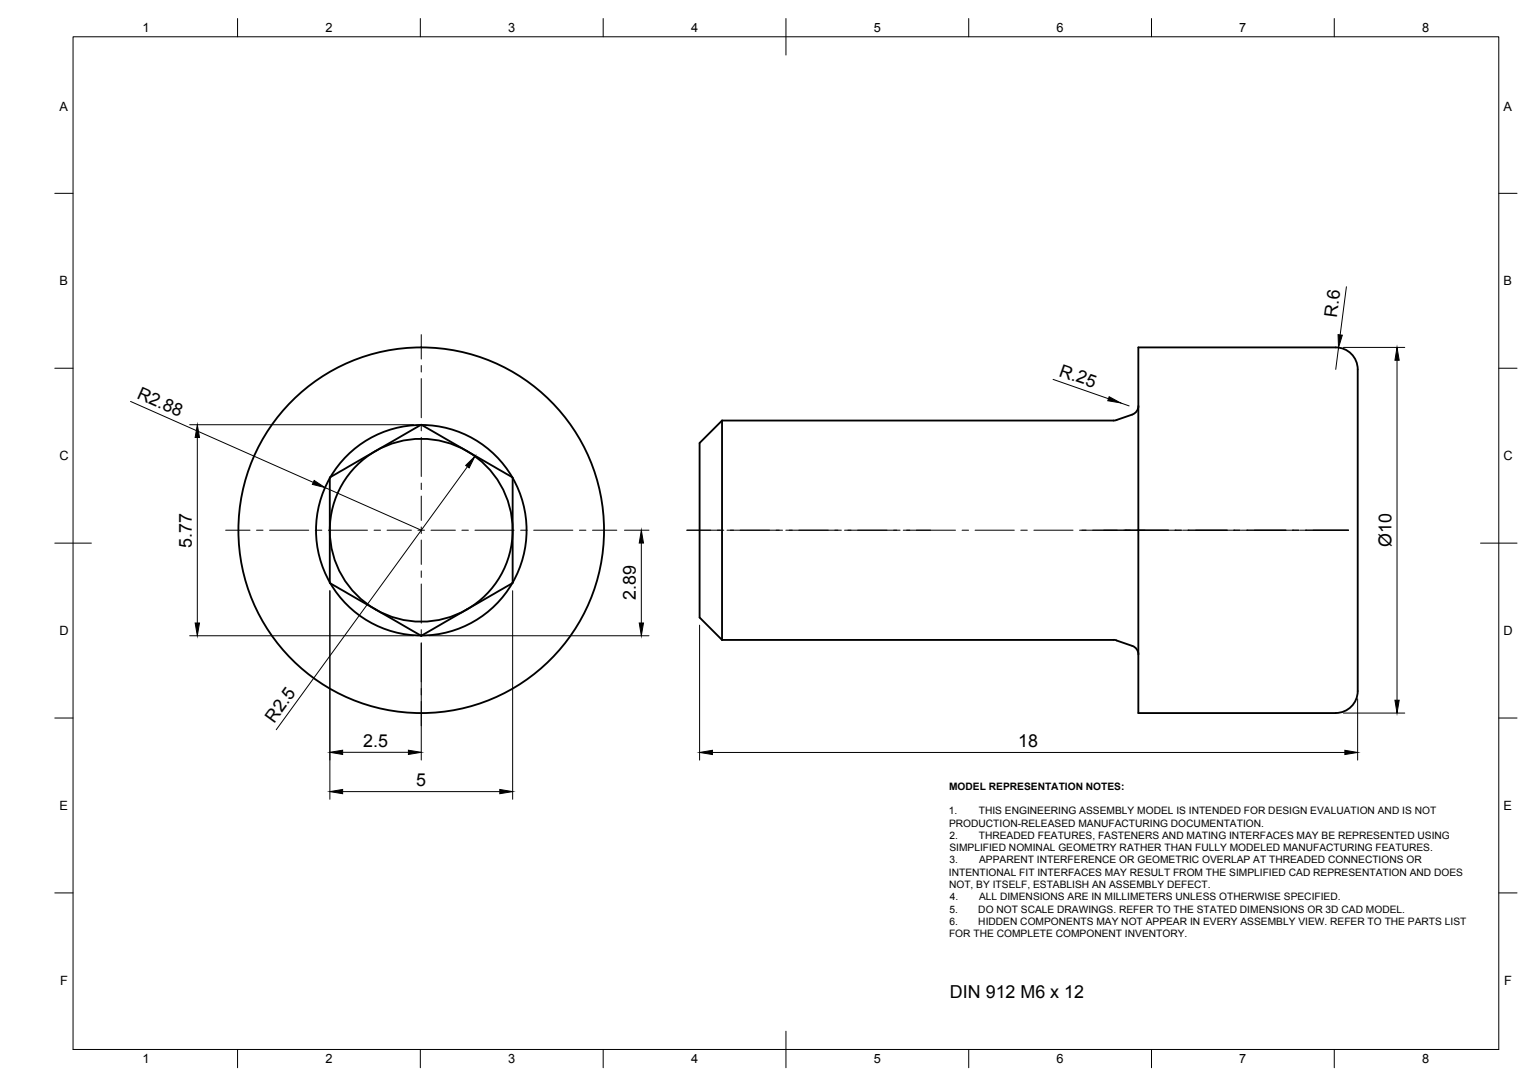
ISO-10303-21;
HEADER;
/* Generated by software containing ST-Developer
 * from STEP Tools, Inc. (www.steptools.com) 
 */

FILE_DESCRIPTION(
/* description */ ('STEP AP214'),
/* implementation_level */ '2;1');

FILE_NAME(
/* name */ 'DIN 912 M6x12.step',
/* time_stamp */ '2026-10-07T12:18:07-07:00',
/* author */ (''),
/* organization */ (''),
/* preprocessor_version */ 'ST-DEVELOPER v20.2',
/* originating_system */ 'Autodesk Translation Framework v15.15.0.0',
/* authorisation */ '');

FILE_SCHEMA (('AUTOMOTIVE_DESIGN { 1 0 10303 214 3 1 1 }'));
ENDSEC;

DATA;
#10=MECHANICAL_DESIGN_GEOMETRIC_PRESENTATION_REPRESENTATION('',(#133),#62974);
#73=(
BOUNDED_CURVE()
B_SPLINE_CURVE(2,(#62798,#62799,#62800),.UNSPECIFIED.,.F.,.F.)
B_SPLINE_CURVE_WITH_KNOTS((3,3),(-0.604448710450841,-0.208150383555822),
 .UNSPECIFIED.)
CURVE()
GEOMETRIC_REPRESENTATION_ITEM()
RATIONAL_B_SPLINE_CURVE((1.32194252928783,1.52287779373958,1.32194252928783))
REPRESENTATION_ITEM('')
);
#74=(
BOUNDED_CURVE()
B_SPLINE_CURVE(2,(#62844,#62845,#62846),.UNSPECIFIED.,.F.,.F.)
B_SPLINE_CURVE_WITH_KNOTS((3,3),(0.208150383555825,0.60444871045084),
 .UNSPECIFIED.)
CURVE()
GEOMETRIC_REPRESENTATION_ITEM()
RATIONAL_B_SPLINE_CURVE((1.32194252928783,1.52287779373957,1.32194252928783))
REPRESENTATION_ITEM('')
);
#75=(
BOUNDED_CURVE()
B_SPLINE_CURVE(2,(#62851,#62852,#62853),.UNSPECIFIED.,.F.,.F.)
B_SPLINE_CURVE_WITH_KNOTS((3,3),(0.208150383555826,0.604448710450838),
 .UNSPECIFIED.)
CURVE()
GEOMETRIC_REPRESENTATION_ITEM()
RATIONAL_B_SPLINE_CURVE((1.32194252928783,1.52287779373957,1.32194252928783))
REPRESENTATION_ITEM('')
);
#76=(
BOUNDED_CURVE()
B_SPLINE_CURVE(2,(#62858,#62859,#62860),.UNSPECIFIED.,.F.,.F.)
B_SPLINE_CURVE_WITH_KNOTS((3,3),(0.208150383555825,0.60444871045084),
 .UNSPECIFIED.)
CURVE()
GEOMETRIC_REPRESENTATION_ITEM()
RATIONAL_B_SPLINE_CURVE((1.32194252928783,1.52287779373957,1.32194252928783))
REPRESENTATION_ITEM('')
);
#77=(
BOUNDED_CURVE()
B_SPLINE_CURVE(2,(#62869,#62870,#62871),.UNSPECIFIED.,.F.,.F.)
B_SPLINE_CURVE_WITH_KNOTS((3,3),(0.208150383555823,0.604448710450839),
 .UNSPECIFIED.)
CURVE()
GEOMETRIC_REPRESENTATION_ITEM()
RATIONAL_B_SPLINE_CURVE((1.32194252928783,1.52287779373958,1.32194252928783))
REPRESENTATION_ITEM('')
);
#78=(
BOUNDED_CURVE()
B_SPLINE_CURVE(2,(#62876,#62877,#62878),.UNSPECIFIED.,.F.,.F.)
B_SPLINE_CURVE_WITH_KNOTS((3,3),(0.208150383555823,0.604448710450836),
 .UNSPECIFIED.)
CURVE()
GEOMETRIC_REPRESENTATION_ITEM()
RATIONAL_B_SPLINE_CURVE((1.32194252928783,1.52287779373958,1.32194252928783))
REPRESENTATION_ITEM('')
);
#109=SHAPE_REPRESENTATION_RELATIONSHIP('SRR','None',#63032,#121);
#121=ADVANCED_BREP_SHAPE_REPRESENTATION('',(#145),#62973);
#133=STYLED_ITEM('',(#63090),#145);
#145=MANIFOLD_SOLID_BREP('Body1',#15203);
#277=FACE_BOUND('',#5497,.T.);
#278=FACE_BOUND('',#5507,.T.);
#720=PLANE('',#16916);
#721=PLANE('',#16923);
#722=PLANE('',#16928);
#723=PLANE('',#16929);
#724=PLANE('',#16930);
#725=PLANE('',#16931);
#726=PLANE('',#16932);
#727=PLANE('',#16933);
#728=PLANE('',#16934);
#729=PLANE('',#16935);
#730=PLANE('',#16936);
#731=PLANE('',#16937);
#732=PLANE('',#16938);
#733=PLANE('',#16939);
#734=PLANE('',#16940);
#1048=CONICAL_SURFACE('',#16885,2.5,1.04719755119659);
#1049=CONICAL_SURFACE('',#16892,2.88,1.04719755119651);
#1050=CONICAL_SURFACE('',#16913,3.,0.785398163397449);
#1051=CONICAL_SURFACE('',#16915,3.0139499546386,0.335638550327472);
#1052=CONICAL_SURFACE('',#16917,2.88,1.04719755119651);
#1053=CONICAL_SURFACE('',#16919,2.88,1.04719755119651);
#1054=CONICAL_SURFACE('',#16921,2.88,1.04719755119651);
#1055=CONICAL_SURFACE('',#16924,2.88,1.04719755119651);
#1056=CONICAL_SURFACE('',#16926,2.88,1.04719755119651);
#2215=LINE('',#62783,#3408);
#2216=LINE('',#62812,#3409);
#2217=LINE('',#62824,#3410);
#2218=LINE('',#62836,#3411);
#2219=LINE('',#62839,#3412);
#2220=LINE('',#62864,#3413);
#2221=LINE('',#62865,#3414);
#2222=LINE('',#62882,#3415);
#2223=LINE('',#62883,#3416);
#2224=LINE('',#62886,#3417);
#2225=LINE('',#62887,#3418);
#2226=LINE('',#62891,#3419);
#2227=LINE('',#62892,#3420);
#2228=LINE('',#62894,#3421);
#2229=LINE('',#62895,#3422);
#2230=LINE('',#62897,#3423);
#2231=LINE('',#62899,#3424);
#2232=LINE('',#62900,#3425);
#2233=LINE('',#62902,#3426);
#2234=LINE('',#62904,#3427);
#2235=LINE('',#62906,#3428);
#2236=LINE('',#62907,#3429);
#2237=LINE('',#62909,#3430);
#2238=LINE('',#62910,#3431);
#2239=LINE('',#62912,#3432);
#2240=LINE('',#62914,#3433);
#2241=LINE('',#62915,#3434);
#2242=LINE('',#62918,#3435);
#2243=LINE('',#62920,#3436);
#2244=LINE('',#62921,#3437);
#2245=LINE('',#62922,#3438);
#2246=LINE('',#62924,#3439);
#2247=LINE('',#62925,#3440);
#2248=LINE('',#62926,#3441);
#2249=LINE('',#62927,#3442);
#3408=VECTOR('',#21212,2.5);
#3409=VECTOR('',#21241,5.);
#3410=VECTOR('',#21256,3.);
#3411=VECTOR('',#21271,3.);
#3412=VECTOR('',#21276,3.0139499546386);
#3413=VECTOR('',#21293,1000.);
#3414=VECTOR('',#21294,1000.);
#3415=VECTOR('',#21305,1000.);
#3416=VECTOR('',#21306,1000.);
#3417=VECTOR('',#21309,1000.);
#3418=VECTOR('',#21310,1000.);
#3419=VECTOR('',#21315,1000.);
#3420=VECTOR('',#21316,1000.);
#3421=VECTOR('',#21317,1000.);
#3422=VECTOR('',#21318,1000.);
#3423=VECTOR('',#21321,1000.);
#3424=VECTOR('',#21322,1000.);
#3425=VECTOR('',#21323,1000.);
#3426=VECTOR('',#21326,1000.);
#3427=VECTOR('',#21327,1000.);
#3428=VECTOR('',#21328,1000.);
#3429=VECTOR('',#21329,1000.);
#3430=VECTOR('',#21332,1000.);
#3431=VECTOR('',#21333,1000.);
#3432=VECTOR('',#21334,1000.);
#3433=VECTOR('',#21335,1000.);
#3434=VECTOR('',#21336,1000.);
#3435=VECTOR('',#21339,1000.);
#3436=VECTOR('',#21340,1000.);
#3437=VECTOR('',#21341,1000.);
#3438=VECTOR('',#21342,1000.);
#3439=VECTOR('',#21345,1000.);
#3440=VECTOR('',#21346,1000.);
#3441=VECTOR('',#21347,1000.);
#3442=VECTOR('',#21348,1000.);
#3688=CYLINDRICAL_SURFACE('',#16899,5.);
#3689=CYLINDRICAL_SURFACE('',#16906,3.);
#4528=FACE_OUTER_BOUND('',#5478,.T.);
#4529=FACE_OUTER_BOUND('',#5479,.T.);
#4530=FACE_OUTER_BOUND('',#5480,.T.);
#4531=FACE_OUTER_BOUND('',#5481,.T.);
#4532=FACE_OUTER_BOUND('',#5482,.T.);
#4533=FACE_OUTER_BOUND('',#5483,.T.);
#4534=FACE_OUTER_BOUND('',#5484,.T.);
#4535=FACE_OUTER_BOUND('',#5485,.T.);
#4536=FACE_OUTER_BOUND('',#5486,.T.);
#4537=FACE_OUTER_BOUND('',#5487,.T.);
#4538=FACE_OUTER_BOUND('',#5488,.T.);
#4539=FACE_OUTER_BOUND('',#5489,.T.);
#4540=FACE_OUTER_BOUND('',#5490,.T.);
#4541=FACE_OUTER_BOUND('',#5491,.T.);
#4542=FACE_OUTER_BOUND('',#5492,.T.);
#4543=FACE_OUTER_BOUND('',#5493,.T.);
#4544=FACE_OUTER_BOUND('',#5494,.T.);
#4545=FACE_OUTER_BOUND('',#5495,.T.);
#4546=FACE_OUTER_BOUND('',#5496,.T.);
#4547=FACE_OUTER_BOUND('',#5498,.T.);
#4548=FACE_OUTER_BOUND('',#5499,.T.);
#4549=FACE_OUTER_BOUND('',#5500,.T.);
#4550=FACE_OUTER_BOUND('',#5501,.T.);
#4551=FACE_OUTER_BOUND('',#5502,.T.);
#4552=FACE_OUTER_BOUND('',#5503,.T.);
#4553=FACE_OUTER_BOUND('',#5504,.T.);
#4554=FACE_OUTER_BOUND('',#5505,.T.);
#4555=FACE_OUTER_BOUND('',#5506,.T.);
#4556=FACE_OUTER_BOUND('',#5508,.T.);
#5478=EDGE_LOOP('',(#14117,#14118,#14119,#14120,#14121,#14122,#14123,#14124));
#5479=EDGE_LOOP('',(#14125,#14126));
#5480=EDGE_LOOP('',(#14127,#14128,#14129,#14130,#14131));
#5481=EDGE_LOOP('',(#14132,#14133,#14134,#14135,#14136));
#5482=EDGE_LOOP('',(#14137,#14138,#14139,#14140,#14141));
#5483=EDGE_LOOP('',(#14142,#14143,#14144,#14145,#14146,#14147));
#5484=EDGE_LOOP('',(#14148,#14149,#14150,#14151));
#5485=EDGE_LOOP('',(#14152,#14153,#14154,#14155,#14156));
#5486=EDGE_LOOP('',(#14157,#14158,#14159,#14160));
#5487=EDGE_LOOP('',(#14161));
#5488=EDGE_LOOP('',(#14162,#14163));
#5489=EDGE_LOOP('',(#14164,#14165));
#5490=EDGE_LOOP('',(#14166,#14167));
#5491=EDGE_LOOP('',(#14168,#14169,#14170));
#5492=EDGE_LOOP('',(#14171,#14172));
#5493=EDGE_LOOP('',(#14173,#14174));
#5494=EDGE_LOOP('',(#14175,#14176,#14177));
#5495=EDGE_LOOP('',(#14178,#14179,#14180));
#5496=EDGE_LOOP('',(#14181));
#5497=EDGE_LOOP('',(#14182));
#5498=EDGE_LOOP('',(#14183,#14184,#14185,#14186,#14187,#14188,#14189));
#5499=EDGE_LOOP('',(#14190,#14191,#14192,#14193,#14194,#14195,#14196));
#5500=EDGE_LOOP('',(#14197,#14198,#14199,#14200,#14201,#14202,#14203));
#5501=EDGE_LOOP('',(#14204,#14205,#14206,#14207,#14208,#14209,#14210));
#5502=EDGE_LOOP('',(#14211,#14212,#14213,#14214,#14215,#14216,#14217));
#5503=EDGE_LOOP('',(#14218,#14219,#14220,#14221,#14222,#14223,#14224));
#5504=EDGE_LOOP('',(#14225,#14226,#14227));
#5505=EDGE_LOOP('',(#14228,#14229,#14230));
#5506=EDGE_LOOP('',(#14231));
#5507=EDGE_LOOP('',(#14232,#14233,#14234,#14235,#14236,#14237,#14238,#14239,
#14240,#14241,#14242,#14243,#14244,#14245,#14246,#14247,#14248,#14249));
#5508=EDGE_LOOP('',(#14250,#14251,#14252));
#6194=CIRCLE('',#16886,2.5);
#6195=CIRCLE('',#16887,2.5);
#6196=CIRCLE('',#16888,2.5);
#6197=CIRCLE('',#16889,2.5);
#6198=CIRCLE('',#16890,2.5);
#6199=CIRCLE('',#16891,2.5);
#6200=CIRCLE('',#16893,2.88);
#6201=CIRCLE('',#16895,4.4);
#6202=CIRCLE('',#16896,0.600000000000098);
#6203=CIRCLE('',#16897,5.);
#6204=CIRCLE('',#16898,5.);
#6205=CIRCLE('',#16900,5.);
#6206=CIRCLE('',#16902,3.0139499546386);
#6207=CIRCLE('',#16903,0.249999999998187);
#6208=CIRCLE('',#16904,3.);
#6209=CIRCLE('',#16905,3.);
#6210=CIRCLE('',#16907,3.);
#6211=CIRCLE('',#16908,3.);
#6212=CIRCLE('',#16910,3.4);
#6213=CIRCLE('',#16911,0.249999999999786);
#6214=CIRCLE('',#16912,3.1639499546386);
#6215=CIRCLE('',#16914,2.3865);
#6216=CIRCLE('',#16918,2.88);
#6217=CIRCLE('',#16920,2.88);
#6218=CIRCLE('',#16922,2.88);
#6219=CIRCLE('',#16925,2.88);
#6220=CIRCLE('',#16927,2.88);
#7580=VERTEX_POINT('',#62781);
#7581=VERTEX_POINT('',#62782);
#7582=VERTEX_POINT('',#62784);
#7583=VERTEX_POINT('',#62786);
#7584=VERTEX_POINT('',#62788);
#7585=VERTEX_POINT('',#62790);
#7586=VERTEX_POINT('',#62792);
#7587=VERTEX_POINT('',#62796);
#7588=VERTEX_POINT('',#62797);
#7589=VERTEX_POINT('',#62803);
#7590=VERTEX_POINT('',#62805);
#7591=VERTEX_POINT('',#62807);
#7592=VERTEX_POINT('',#62811);
#7593=VERTEX_POINT('',#62815);
#7594=VERTEX_POINT('',#62817);
#7595=VERTEX_POINT('',#62819);
#7596=VERTEX_POINT('',#62823);
#7597=VERTEX_POINT('',#62825);
#7598=VERTEX_POINT('',#62829);
#7599=VERTEX_POINT('',#62831);
#7600=VERTEX_POINT('',#62835);
#7601=VERTEX_POINT('',#62842);
#7602=VERTEX_POINT('',#62843);
#7603=VERTEX_POINT('',#62849);
#7604=VERTEX_POINT('',#62850);
#7605=VERTEX_POINT('',#62856);
#7606=VERTEX_POINT('',#62857);
#7607=VERTEX_POINT('',#62863);
#7608=VERTEX_POINT('',#62867);
#7609=VERTEX_POINT('',#62868);
#7610=VERTEX_POINT('',#62874);
#7611=VERTEX_POINT('',#62875);
#7612=VERTEX_POINT('',#62881);
#7613=VERTEX_POINT('',#62885);
#7614=VERTEX_POINT('',#62890);
#7615=VERTEX_POINT('',#62893);
#7616=VERTEX_POINT('',#62898);
#7617=VERTEX_POINT('',#62903);
#7618=VERTEX_POINT('',#62905);
#7619=VERTEX_POINT('',#62911);
#7620=VERTEX_POINT('',#62913);
#7621=VERTEX_POINT('',#62917);
#7622=VERTEX_POINT('',#62919);
#9765=EDGE_CURVE('',#7580,#7581,#2215,.T.);
#9766=EDGE_CURVE('',#7582,#7581,#6194,.T.);
#9767=EDGE_CURVE('',#7583,#7582,#6195,.T.);
#9768=EDGE_CURVE('',#7584,#7583,#6196,.T.);
#9769=EDGE_CURVE('',#7585,#7584,#6197,.T.);
#9770=EDGE_CURVE('',#7586,#7585,#6198,.T.);
#9771=EDGE_CURVE('',#7581,#7586,#6199,.T.);
#9772=EDGE_CURVE('',#7587,#7588,#73,.F.);
#9773=EDGE_CURVE('',#7587,#7588,#6200,.T.);
#9774=EDGE_CURVE('',#7589,#7589,#6201,.T.);
#9775=EDGE_CURVE('',#7589,#7590,#6202,.T.);
#9776=EDGE_CURVE('',#7590,#7591,#6203,.T.);
#9777=EDGE_CURVE('',#7591,#7590,#6204,.T.);
#9778=EDGE_CURVE('',#7591,#7592,#2216,.T.);
#9779=EDGE_CURVE('',#7592,#7592,#6205,.T.);
#9780=EDGE_CURVE('',#7593,#7593,#6206,.T.);
#9781=EDGE_CURVE('',#7593,#7594,#6207,.T.);
#9782=EDGE_CURVE('',#7594,#7595,#6208,.T.);
#9783=EDGE_CURVE('',#7595,#7594,#6209,.T.);
#9784=EDGE_CURVE('',#7595,#7596,#2217,.T.);
#9785=EDGE_CURVE('',#7597,#7596,#6210,.T.);
#9786=EDGE_CURVE('',#7596,#7597,#6211,.T.);
#9787=EDGE_CURVE('',#7598,#7598,#6212,.T.);
#9788=EDGE_CURVE('',#7598,#7599,#6213,.T.);
#9789=EDGE_CURVE('',#7599,#7599,#6214,.T.);
#9790=EDGE_CURVE('',#7597,#7600,#2218,.T.);
#9791=EDGE_CURVE('',#7600,#7600,#6215,.T.);
#9792=EDGE_CURVE('',#7599,#7593,#2219,.T.);
#9793=EDGE_CURVE('',#7601,#7602,#74,.T.);
#9794=EDGE_CURVE('',#7601,#7602,#6216,.T.);
#9795=EDGE_CURVE('',#7603,#7604,#75,.T.);
#9796=EDGE_CURVE('',#7603,#7604,#6217,.T.);
#9797=EDGE_CURVE('',#7605,#7606,#76,.T.);
#9798=EDGE_CURVE('',#7605,#7606,#6218,.T.);
#9799=EDGE_CURVE('',#7585,#7607,#2220,.T.);
#9800=EDGE_CURVE('',#7607,#7584,#2221,.T.);
#9801=EDGE_CURVE('',#7608,#7609,#77,.T.);
#9802=EDGE_CURVE('',#7608,#7609,#6219,.T.);
#9803=EDGE_CURVE('',#7610,#7611,#78,.T.);
#9804=EDGE_CURVE('',#7610,#7611,#6220,.T.);
#9805=EDGE_CURVE('',#7584,#7612,#2222,.T.);
#9806=EDGE_CURVE('',#7612,#7583,#2223,.T.);
#9807=EDGE_CURVE('',#7583,#7613,#2224,.T.);
#9808=EDGE_CURVE('',#7613,#7582,#2225,.T.);
#9809=EDGE_CURVE('',#7614,#7588,#2226,.T.);
#9810=EDGE_CURVE('',#7607,#7614,#2227,.T.);
#9811=EDGE_CURVE('',#7612,#7615,#2228,.T.);
#9812=EDGE_CURVE('',#7615,#7587,#2229,.T.);
#9813=EDGE_CURVE('',#7615,#7611,#2230,.T.);
#9814=EDGE_CURVE('',#7613,#7616,#2231,.T.);
#9815=EDGE_CURVE('',#7616,#7610,#2232,.T.);
#9816=EDGE_CURVE('',#7616,#7606,#2233,.T.);
#9817=EDGE_CURVE('',#7582,#7617,#2234,.T.);
#9818=EDGE_CURVE('',#7617,#7618,#2235,.T.);
#9819=EDGE_CURVE('',#7618,#7605,#2236,.T.);
#9820=EDGE_CURVE('',#7618,#7602,#2237,.T.);
#9821=EDGE_CURVE('',#7617,#7581,#2238,.T.);
#9822=EDGE_CURVE('',#7581,#7619,#2239,.T.);
#9823=EDGE_CURVE('',#7619,#7620,#2240,.T.);
#9824=EDGE_CURVE('',#7620,#7601,#2241,.T.);
#9825=EDGE_CURVE('',#7621,#7609,#2242,.T.);
#9826=EDGE_CURVE('',#7622,#7621,#2243,.T.);
#9827=EDGE_CURVE('',#7622,#7585,#2244,.T.);
#9828=EDGE_CURVE('',#7614,#7608,#2245,.T.);
#9829=EDGE_CURVE('',#7620,#7604,#2246,.T.);
#9830=EDGE_CURVE('',#7619,#7586,#2247,.T.);
#9831=EDGE_CURVE('',#7586,#7622,#2248,.T.);
#9832=EDGE_CURVE('',#7621,#7603,#2249,.T.);
#14117=ORIENTED_EDGE('',*,*,#9765,.T.);
#14118=ORIENTED_EDGE('',*,*,#9766,.F.);
#14119=ORIENTED_EDGE('',*,*,#9767,.F.);
#14120=ORIENTED_EDGE('',*,*,#9768,.F.);
#14121=ORIENTED_EDGE('',*,*,#9769,.F.);
#14122=ORIENTED_EDGE('',*,*,#9770,.F.);
#14123=ORIENTED_EDGE('',*,*,#9771,.F.);
#14124=ORIENTED_EDGE('',*,*,#9765,.F.);
#14125=ORIENTED_EDGE('',*,*,#9772,.F.);
#14126=ORIENTED_EDGE('',*,*,#9773,.T.);
#14127=ORIENTED_EDGE('',*,*,#9774,.F.);
#14128=ORIENTED_EDGE('',*,*,#9775,.T.);
#14129=ORIENTED_EDGE('',*,*,#9776,.T.);
#14130=ORIENTED_EDGE('',*,*,#9777,.T.);
#14131=ORIENTED_EDGE('',*,*,#9775,.F.);
#14132=ORIENTED_EDGE('',*,*,#9777,.F.);
#14133=ORIENTED_EDGE('',*,*,#9778,.T.);
#14134=ORIENTED_EDGE('',*,*,#9779,.F.);
#14135=ORIENTED_EDGE('',*,*,#9778,.F.);
#14136=ORIENTED_EDGE('',*,*,#9776,.F.);
#14137=ORIENTED_EDGE('',*,*,#9780,.F.);
#14138=ORIENTED_EDGE('',*,*,#9781,.T.);
#14139=ORIENTED_EDGE('',*,*,#9782,.T.);
#14140=ORIENTED_EDGE('',*,*,#9783,.T.);
#14141=ORIENTED_EDGE('',*,*,#9781,.F.);
#14142=ORIENTED_EDGE('',*,*,#9783,.F.);
#14143=ORIENTED_EDGE('',*,*,#9784,.T.);
#14144=ORIENTED_EDGE('',*,*,#9785,.F.);
#14145=ORIENTED_EDGE('',*,*,#9786,.F.);
#14146=ORIENTED_EDGE('',*,*,#9784,.F.);
#14147=ORIENTED_EDGE('',*,*,#9782,.F.);
#14148=ORIENTED_EDGE('',*,*,#9787,.F.);
#14149=ORIENTED_EDGE('',*,*,#9788,.T.);
#14150=ORIENTED_EDGE('',*,*,#9789,.T.);
#14151=ORIENTED_EDGE('',*,*,#9788,.F.);
#14152=ORIENTED_EDGE('',*,*,#9785,.T.);
#14153=ORIENTED_EDGE('',*,*,#9786,.T.);
#14154=ORIENTED_EDGE('',*,*,#9790,.T.);
#14155=ORIENTED_EDGE('',*,*,#9791,.F.);
#14156=ORIENTED_EDGE('',*,*,#9790,.F.);
#14157=ORIENTED_EDGE('',*,*,#9789,.F.);
#14158=ORIENTED_EDGE('',*,*,#9792,.T.);
#14159=ORIENTED_EDGE('',*,*,#9780,.T.);
#14160=ORIENTED_EDGE('',*,*,#9792,.F.);
#14161=ORIENTED_EDGE('',*,*,#9791,.T.);
#14162=ORIENTED_EDGE('',*,*,#9793,.F.);
#14163=ORIENTED_EDGE('',*,*,#9794,.T.);
#14164=ORIENTED_EDGE('',*,*,#9795,.F.);
#14165=ORIENTED_EDGE('',*,*,#9796,.T.);
#14166=ORIENTED_EDGE('',*,*,#9797,.F.);
#14167=ORIENTED_EDGE('',*,*,#9798,.T.);
#14168=ORIENTED_EDGE('',*,*,#9799,.F.);
#14169=ORIENTED_EDGE('',*,*,#9769,.T.);
#14170=ORIENTED_EDGE('',*,*,#9800,.F.);
#14171=ORIENTED_EDGE('',*,*,#9801,.F.);
#14172=ORIENTED_EDGE('',*,*,#9802,.T.);
#14173=ORIENTED_EDGE('',*,*,#9803,.F.);
#14174=ORIENTED_EDGE('',*,*,#9804,.T.);
#14175=ORIENTED_EDGE('',*,*,#9805,.F.);
#14176=ORIENTED_EDGE('',*,*,#9768,.T.);
#14177=ORIENTED_EDGE('',*,*,#9806,.F.);
#14178=ORIENTED_EDGE('',*,*,#9807,.F.);
#14179=ORIENTED_EDGE('',*,*,#9767,.T.);
#14180=ORIENTED_EDGE('',*,*,#9808,.F.);
#14181=ORIENTED_EDGE('',*,*,#9779,.T.);
#14182=ORIENTED_EDGE('',*,*,#9787,.T.);
#14183=ORIENTED_EDGE('',*,*,#9772,.T.);
#14184=ORIENTED_EDGE('',*,*,#9809,.F.);
#14185=ORIENTED_EDGE('',*,*,#9810,.F.);
#14186=ORIENTED_EDGE('',*,*,#9800,.T.);
#14187=ORIENTED_EDGE('',*,*,#9805,.T.);
#14188=ORIENTED_EDGE('',*,*,#9811,.T.);
#14189=ORIENTED_EDGE('',*,*,#9812,.T.);
#14190=ORIENTED_EDGE('',*,*,#9803,.T.);
#14191=ORIENTED_EDGE('',*,*,#9813,.F.);
#14192=ORIENTED_EDGE('',*,*,#9811,.F.);
#14193=ORIENTED_EDGE('',*,*,#9806,.T.);
#14194=ORIENTED_EDGE('',*,*,#9807,.T.);
#14195=ORIENTED_EDGE('',*,*,#9814,.T.);
#14196=ORIENTED_EDGE('',*,*,#9815,.T.);
#14197=ORIENTED_EDGE('',*,*,#9797,.T.);
#14198=ORIENTED_EDGE('',*,*,#9816,.F.);
#14199=ORIENTED_EDGE('',*,*,#9814,.F.);
#14200=ORIENTED_EDGE('',*,*,#9808,.T.);
#14201=ORIENTED_EDGE('',*,*,#9817,.T.);
#14202=ORIENTED_EDGE('',*,*,#9818,.T.);
#14203=ORIENTED_EDGE('',*,*,#9819,.T.);
#14204=ORIENTED_EDGE('',*,*,#9793,.T.);
#14205=ORIENTED_EDGE('',*,*,#9820,.F.);
#14206=ORIENTED_EDGE('',*,*,#9818,.F.);
#14207=ORIENTED_EDGE('',*,*,#9821,.T.);
#14208=ORIENTED_EDGE('',*,*,#9822,.T.);
#14209=ORIENTED_EDGE('',*,*,#9823,.T.);
#14210=ORIENTED_EDGE('',*,*,#9824,.T.);
#14211=ORIENTED_EDGE('',*,*,#9801,.T.);
#14212=ORIENTED_EDGE('',*,*,#9825,.F.);
#14213=ORIENTED_EDGE('',*,*,#9826,.F.);
#14214=ORIENTED_EDGE('',*,*,#9827,.T.);
#14215=ORIENTED_EDGE('',*,*,#9799,.T.);
#14216=ORIENTED_EDGE('',*,*,#9810,.T.);
#14217=ORIENTED_EDGE('',*,*,#9828,.T.);
#14218=ORIENTED_EDGE('',*,*,#9795,.T.);
#14219=ORIENTED_EDGE('',*,*,#9829,.F.);
#14220=ORIENTED_EDGE('',*,*,#9823,.F.);
#14221=ORIENTED_EDGE('',*,*,#9830,.T.);
#14222=ORIENTED_EDGE('',*,*,#9831,.T.);
#14223=ORIENTED_EDGE('',*,*,#9826,.T.);
#14224=ORIENTED_EDGE('',*,*,#9832,.T.);
#14225=ORIENTED_EDGE('',*,*,#9822,.F.);
#14226=ORIENTED_EDGE('',*,*,#9771,.T.);
#14227=ORIENTED_EDGE('',*,*,#9830,.F.);
#14228=ORIENTED_EDGE('',*,*,#9817,.F.);
#14229=ORIENTED_EDGE('',*,*,#9766,.T.);
#14230=ORIENTED_EDGE('',*,*,#9821,.F.);
#14231=ORIENTED_EDGE('',*,*,#9774,.T.);
#14232=ORIENTED_EDGE('',*,*,#9812,.F.);
#14233=ORIENTED_EDGE('',*,*,#9813,.T.);
#14234=ORIENTED_EDGE('',*,*,#9804,.F.);
#14235=ORIENTED_EDGE('',*,*,#9815,.F.);
#14236=ORIENTED_EDGE('',*,*,#9816,.T.);
#14237=ORIENTED_EDGE('',*,*,#9798,.F.);
#14238=ORIENTED_EDGE('',*,*,#9819,.F.);
#14239=ORIENTED_EDGE('',*,*,#9820,.T.);
#14240=ORIENTED_EDGE('',*,*,#9794,.F.);
#14241=ORIENTED_EDGE('',*,*,#9824,.F.);
#14242=ORIENTED_EDGE('',*,*,#9829,.T.);
#14243=ORIENTED_EDGE('',*,*,#9796,.F.);
#14244=ORIENTED_EDGE('',*,*,#9832,.F.);
#14245=ORIENTED_EDGE('',*,*,#9825,.T.);
#14246=ORIENTED_EDGE('',*,*,#9802,.F.);
#14247=ORIENTED_EDGE('',*,*,#9828,.F.);
#14248=ORIENTED_EDGE('',*,*,#9809,.T.);
#14249=ORIENTED_EDGE('',*,*,#9773,.F.);
#14250=ORIENTED_EDGE('',*,*,#9831,.F.);
#14251=ORIENTED_EDGE('',*,*,#9770,.T.);
#14252=ORIENTED_EDGE('',*,*,#9827,.F.);
#14322=TOROIDAL_SURFACE('',#16894,4.39999999999991,0.600000000000098);
#14323=TOROIDAL_SURFACE('',#16901,3.24999999999819,0.249999999998187);
#14324=TOROIDAL_SURFACE('',#16909,3.39999999999989,0.249999999999786);
#15163=ADVANCED_FACE('',(#4528),#1048,.F.);
#15164=ADVANCED_FACE('',(#4529),#1049,.F.);
#15165=ADVANCED_FACE('',(#4530),#14322,.T.);
#15166=ADVANCED_FACE('',(#4531),#3688,.T.);
#15167=ADVANCED_FACE('',(#4532),#14323,.F.);
#15168=ADVANCED_FACE('',(#4533),#3689,.T.);
#15169=ADVANCED_FACE('',(#4534),#14324,.F.);
#15170=ADVANCED_FACE('',(#4535),#1050,.T.);
#15171=ADVANCED_FACE('',(#4536),#1051,.T.);
#15172=ADVANCED_FACE('',(#4537),#720,.F.);
#15173=ADVANCED_FACE('',(#4538),#1052,.F.);
#15174=ADVANCED_FACE('',(#4539),#1053,.F.);
#15175=ADVANCED_FACE('',(#4540),#1054,.F.);
#15176=ADVANCED_FACE('',(#4541),#721,.F.);
#15177=ADVANCED_FACE('',(#4542),#1055,.F.);
#15178=ADVANCED_FACE('',(#4543),#1056,.F.);
#15179=ADVANCED_FACE('',(#4544),#722,.F.);
#15180=ADVANCED_FACE('',(#4545),#723,.F.);
#15181=ADVANCED_FACE('',(#4546,#277),#724,.F.);
#15182=ADVANCED_FACE('',(#4547),#725,.T.);
#15183=ADVANCED_FACE('',(#4548),#726,.T.);
#15184=ADVANCED_FACE('',(#4549),#727,.T.);
#15185=ADVANCED_FACE('',(#4550),#728,.T.);
#15186=ADVANCED_FACE('',(#4551),#729,.T.);
#15187=ADVANCED_FACE('',(#4552),#730,.T.);
#15188=ADVANCED_FACE('',(#4553),#731,.F.);
#15189=ADVANCED_FACE('',(#4554),#732,.F.);
#15190=ADVANCED_FACE('',(#4555,#278),#733,.F.);
#15191=ADVANCED_FACE('',(#4556),#734,.F.);
#15203=CLOSED_SHELL('',(#15163,#15164,#15165,#15166,#15167,#15168,#15169,
#15170,#15171,#15172,#15173,#15174,#15175,#15176,#15177,#15178,#15179,#15180,
#15181,#15182,#15183,#15184,#15185,#15186,#15187,#15188,#15189,#15190,#15191));
#16884=AXIS2_PLACEMENT_3D('',#62779,#21208,#21209);
#16885=AXIS2_PLACEMENT_3D('',#62780,#21210,#21211);
#16886=AXIS2_PLACEMENT_3D('',#62785,#21213,#21214);
#16887=AXIS2_PLACEMENT_3D('',#62787,#21215,#21216);
#16888=AXIS2_PLACEMENT_3D('',#62789,#21217,#21218);
#16889=AXIS2_PLACEMENT_3D('',#62791,#21219,#21220);
#16890=AXIS2_PLACEMENT_3D('',#62793,#21221,#21222);
#16891=AXIS2_PLACEMENT_3D('',#62794,#21223,#21224);
#16892=AXIS2_PLACEMENT_3D('',#62795,#21225,#21226);
#16893=AXIS2_PLACEMENT_3D('',#62801,#21227,#21228);
#16894=AXIS2_PLACEMENT_3D('',#62802,#21229,#21230);
#16895=AXIS2_PLACEMENT_3D('',#62804,#21231,#21232);
#16896=AXIS2_PLACEMENT_3D('',#62806,#21233,#21234);
#16897=AXIS2_PLACEMENT_3D('',#62808,#21235,#21236);
#16898=AXIS2_PLACEMENT_3D('',#62809,#21237,#21238);
#16899=AXIS2_PLACEMENT_3D('',#62810,#21239,#21240);
#16900=AXIS2_PLACEMENT_3D('',#62813,#21242,#21243);
#16901=AXIS2_PLACEMENT_3D('',#62814,#21244,#21245);
#16902=AXIS2_PLACEMENT_3D('',#62816,#21246,#21247);
#16903=AXIS2_PLACEMENT_3D('',#62818,#21248,#21249);
#16904=AXIS2_PLACEMENT_3D('',#62820,#21250,#21251);
#16905=AXIS2_PLACEMENT_3D('',#62821,#21252,#21253);
#16906=AXIS2_PLACEMENT_3D('',#62822,#21254,#21255);
#16907=AXIS2_PLACEMENT_3D('',#62826,#21257,#21258);
#16908=AXIS2_PLACEMENT_3D('',#62827,#21259,#21260);
#16909=AXIS2_PLACEMENT_3D('',#62828,#21261,#21262);
#16910=AXIS2_PLACEMENT_3D('',#62830,#21263,#21264);
#16911=AXIS2_PLACEMENT_3D('',#62832,#21265,#21266);
#16912=AXIS2_PLACEMENT_3D('',#62833,#21267,#21268);
#16913=AXIS2_PLACEMENT_3D('',#62834,#21269,#21270);
#16914=AXIS2_PLACEMENT_3D('',#62837,#21272,#21273);
#16915=AXIS2_PLACEMENT_3D('',#62838,#21274,#21275);
#16916=AXIS2_PLACEMENT_3D('',#62840,#21277,#21278);
#16917=AXIS2_PLACEMENT_3D('',#62841,#21279,#21280);
#16918=AXIS2_PLACEMENT_3D('',#62847,#21281,#21282);
#16919=AXIS2_PLACEMENT_3D('',#62848,#21283,#21284);
#16920=AXIS2_PLACEMENT_3D('',#62854,#21285,#21286);
#16921=AXIS2_PLACEMENT_3D('',#62855,#21287,#21288);
#16922=AXIS2_PLACEMENT_3D('',#62861,#21289,#21290);
#16923=AXIS2_PLACEMENT_3D('',#62862,#21291,#21292);
#16924=AXIS2_PLACEMENT_3D('',#62866,#21295,#21296);
#16925=AXIS2_PLACEMENT_3D('',#62872,#21297,#21298);
#16926=AXIS2_PLACEMENT_3D('',#62873,#21299,#21300);
#16927=AXIS2_PLACEMENT_3D('',#62879,#21301,#21302);
#16928=AXIS2_PLACEMENT_3D('',#62880,#21303,#21304);
#16929=AXIS2_PLACEMENT_3D('',#62884,#21307,#21308);
#16930=AXIS2_PLACEMENT_3D('',#62888,#21311,#21312);
#16931=AXIS2_PLACEMENT_3D('',#62889,#21313,#21314);
#16932=AXIS2_PLACEMENT_3D('',#62896,#21319,#21320);
#16933=AXIS2_PLACEMENT_3D('',#62901,#21324,#21325);
#16934=AXIS2_PLACEMENT_3D('',#62908,#21330,#21331);
#16935=AXIS2_PLACEMENT_3D('',#62916,#21337,#21338);
#16936=AXIS2_PLACEMENT_3D('',#62923,#21343,#21344);
#16937=AXIS2_PLACEMENT_3D('',#62928,#21349,#21350);
#16938=AXIS2_PLACEMENT_3D('',#62929,#21351,#21352);
#16939=AXIS2_PLACEMENT_3D('',#62930,#21353,#21354);
#16940=AXIS2_PLACEMENT_3D('',#62931,#21355,#21356);
#21208=DIRECTION('axis',(0.,0.,1.));
#21209=DIRECTION('refdir',(1.,0.,0.));
#21210=DIRECTION('center_axis',(0.,-1.,-1.E-15));
#21211=DIRECTION('ref_axis',(0.,-1.E-15,1.));
#21212=DIRECTION('',(1.0605752387249E-16,-0.500000000000006,-0.866025403784435));
#21213=DIRECTION('center_axis',(0.,1.,1.E-15));
#21214=DIRECTION('ref_axis',(0.,1.E-15,-1.));
#21215=DIRECTION('center_axis',(0.,1.,1.E-15));
#21216=DIRECTION('ref_axis',(0.,1.E-15,-1.));
#21217=DIRECTION('center_axis',(0.,1.,1.E-15));
#21218=DIRECTION('ref_axis',(0.,1.E-15,-1.));
#21219=DIRECTION('center_axis',(0.,1.,1.E-15));
#21220=DIRECTION('ref_axis',(0.,1.E-15,-1.));
#21221=DIRECTION('center_axis',(0.,1.,1.E-15));
#21222=DIRECTION('ref_axis',(0.,1.E-15,-1.));
#21223=DIRECTION('center_axis',(0.,1.,1.E-15));
#21224=DIRECTION('ref_axis',(0.,1.E-15,-1.));
#21225=DIRECTION('center_axis',(0.,-1.,-1.E-15));
#21226=DIRECTION('ref_axis',(0.,-1.E-15,1.));
#21227=DIRECTION('center_axis',(0.,-1.,-1.E-15));
#21228=DIRECTION('ref_axis',(0.,-1.E-15,1.));
#21229=DIRECTION('center_axis',(0.,-1.,-1.E-15));
#21230=DIRECTION('ref_axis',(0.,-1.4210854715202E-15,1.));
#21231=DIRECTION('center_axis',(0.,-1.,-1.E-15));
#21232=DIRECTION('ref_axis',(0.,-1.E-15,1.));
#21233=DIRECTION('center_axis',(1.,-1.22464678641072E-31,1.22464678641072E-16));
#21234=DIRECTION('ref_axis',(1.22464678641072E-16,1.77635683940025E-15,
-1.));
#21235=DIRECTION('center_axis',(0.,-1.,-1.E-15));
#21236=DIRECTION('ref_axis',(0.,-1.E-15,1.));
#21237=DIRECTION('center_axis',(0.,-1.,-1.E-15));
#21238=DIRECTION('ref_axis',(0.,-1.E-15,1.));
#21239=DIRECTION('center_axis',(0.,-1.,-1.E-15));
#21240=DIRECTION('ref_axis',(0.,1.E-15,-1.));
#21241=DIRECTION('',(0.,1.,1.E-15));
#21242=DIRECTION('center_axis',(0.,1.,1.E-15));
#21243=DIRECTION('ref_axis',(0.,1.E-15,-1.));
#21244=DIRECTION('center_axis',(0.,-1.,-1.E-15));
#21245=DIRECTION('ref_axis',(0.,0.,1.));
#21246=DIRECTION('center_axis',(0.,-1.,-1.E-15));
#21247=DIRECTION('ref_axis',(0.,-1.E-15,1.));
#21248=DIRECTION('center_axis',(-1.,1.22464675805151E-31,-1.22464675805151E-16));
#21249=DIRECTION('ref_axis',(1.22464675805151E-16,0.,-1.));
#21250=DIRECTION('center_axis',(0.,-1.,-1.E-15));
#21251=DIRECTION('ref_axis',(0.,1.E-15,-1.));
#21252=DIRECTION('center_axis',(0.,-1.,-1.E-15));
#21253=DIRECTION('ref_axis',(0.,1.E-15,-1.));
#21254=DIRECTION('center_axis',(0.,-1.,-1.E-15));
#21255=DIRECTION('ref_axis',(0.,1.E-15,-1.));
#21256=DIRECTION('',(0.,1.,1.E-15));
#21257=DIRECTION('center_axis',(0.,1.,1.E-15));
#21258=DIRECTION('ref_axis',(0.,1.E-15,-1.));
#21259=DIRECTION('center_axis',(0.,1.,1.E-15));
#21260=DIRECTION('ref_axis',(0.,1.E-15,-1.));
#21261=DIRECTION('center_axis',(0.,-1.,-1.E-15));
#21262=DIRECTION('ref_axis',(0.,0.,1.));
#21263=DIRECTION('center_axis',(0.,-1.,-1.E-15));
#21264=DIRECTION('ref_axis',(0.,-1.E-15,1.));
#21265=DIRECTION('center_axis',(-1.,1.22464683445529E-31,-1.22464683445529E-16));
#21266=DIRECTION('ref_axis',(1.22464683445529E-16,0.,-1.));
#21267=DIRECTION('center_axis',(0.,-1.,-1.E-15));
#21268=DIRECTION('ref_axis',(0.,-1.E-15,1.));
#21269=DIRECTION('center_axis',(0.,-1.,-1.E-15));
#21270=DIRECTION('ref_axis',(0.,-1.E-15,1.));
#21271=DIRECTION('',(-8.65956056235494E-17,0.707106781186546,0.707106781186549));
#21272=DIRECTION('center_axis',(0.,1.,1.E-15));
#21273=DIRECTION('ref_axis',(0.,1.E-15,-1.));
#21274=DIRECTION('center_axis',(0.,-1.,-1.E-15));
#21275=DIRECTION('ref_axis',(0.,-1.E-15,1.));
#21276=DIRECTION('',(-4.03364556963302E-17,0.944200181445821,0.329372156318165));
#21277=DIRECTION('center_axis',(0.,-1.,-1.E-15));
#21278=DIRECTION('ref_axis',(0.,-1.E-15,1.));
#21279=DIRECTION('center_axis',(0.,-1.,-1.E-15));
#21280=DIRECTION('ref_axis',(1.22464679914735E-16,1.E-15,-1.));
#21281=DIRECTION('center_axis',(0.,-1.,-1.E-15));
#21282=DIRECTION('ref_axis',(0.,-1.E-15,1.));
#21283=DIRECTION('center_axis',(0.,-1.,-1.E-15));
#21284=DIRECTION('ref_axis',(0.,-1.E-15,1.));
#21285=DIRECTION('center_axis',(0.,-1.,-1.E-15));
#21286=DIRECTION('ref_axis',(0.,-1.E-15,1.));
#21287=DIRECTION('center_axis',(0.,-1.,-1.E-15));
#21288=DIRECTION('ref_axis',(0.,-1.E-15,1.));
#21289=DIRECTION('center_axis',(0.,-1.,-1.E-15));
#21290=DIRECTION('ref_axis',(0.,-1.E-15,1.));
#21291=DIRECTION('center_axis',(0.,1.,1.E-15));
#21292=DIRECTION('ref_axis',(-1.,0.,0.));
#21293=DIRECTION('',(0.499999999999983,-8.96640562630007E-16,0.866025403784448));
#21294=DIRECTION('',(1.,-6.12303176911189E-17,-6.12303176911189E-32));
#21295=DIRECTION('center_axis',(0.,-1.,-1.E-15));
#21296=DIRECTION('ref_axis',(0.,-1.E-15,1.));
#21297=DIRECTION('center_axis',(0.,-1.,-1.E-15));
#21298=DIRECTION('ref_axis',(0.,-1.E-15,1.));
#21299=DIRECTION('center_axis',(0.,-1.,-1.E-15));
#21300=DIRECTION('ref_axis',(0.,-1.E-15,1.));
#21301=DIRECTION('center_axis',(0.,-1.,-1.E-15));
#21302=DIRECTION('ref_axis',(0.,-1.E-15,1.));
#21303=DIRECTION('center_axis',(0.,1.,1.E-15));
#21304=DIRECTION('ref_axis',(-1.,0.,0.));
#21305=DIRECTION('',(1.,-6.12303176911189E-17,-6.12303176911189E-32));
#21306=DIRECTION('',(0.499999999999983,8.3541024493889E-16,-0.866025403784448));
#21307=DIRECTION('center_axis',(0.,1.,1.E-15));
#21308=DIRECTION('ref_axis',(-1.,0.,0.));
#21309=DIRECTION('',(0.499999999999983,8.3541024493889E-16,-0.866025403784448));
#21310=DIRECTION('',(-0.499999999999983,8.96640562630007E-16,-0.866025403784448));
#21311=DIRECTION('center_axis',(0.,-1.,-1.E-15));
#21312=DIRECTION('ref_axis',(0.,-1.E-15,1.));
#21313=DIRECTION('center_axis',(0.,1.E-15,-1.));
#21314=DIRECTION('ref_axis',(1.,0.,0.));
#21315=DIRECTION('',(1.,-6.12303176911189E-17,-6.12303176911189E-32));
#21316=DIRECTION('',(0.,-1.,-1.E-15));
#21317=DIRECTION('',(0.,-1.,-1.E-15));
#21318=DIRECTION('',(-1.,0.,0.));
#21319=DIRECTION('center_axis',(-0.866025403784448,4.99999999999983E-16,
-0.499999999999983));
#21320=DIRECTION('ref_axis',(-2.30491487599793E-32,-1.,-1.E-15));
#21321=DIRECTION('',(0.499999999999983,8.3541024493889E-16,-0.866025403784448));
#21322=DIRECTION('',(0.,-1.,-1.E-15));
#21323=DIRECTION('',(-0.499999999999983,-8.66025403784449E-16,0.866025403784448));
#21324=DIRECTION('center_axis',(-0.866025403784448,-4.99999999999983E-16,
0.499999999999983));
#21325=DIRECTION('ref_axis',(-2.30491487599793E-32,1.,1.E-15));
#21326=DIRECTION('',(-0.499999999999983,8.96640562630007E-16,-0.866025403784448));
#21327=DIRECTION('',(-0.499999999999983,8.96640562630007E-16,-0.866025403784448));
#21328=DIRECTION('',(0.,-1.,-1.E-15));
#21329=DIRECTION('',(0.499999999999983,-8.66025403784449E-16,0.866025403784448));
#21330=DIRECTION('center_axis',(0.,-1.E-15,1.));
#21331=DIRECTION('ref_axis',(0.,1.,1.E-15));
#21332=DIRECTION('',(-1.,6.12303176911189E-17,6.12303176911189E-32));
#21333=DIRECTION('',(-1.,6.12303176911189E-17,6.12303176911189E-32));
#21334=DIRECTION('',(-1.,6.12303176911189E-17,6.12303176911189E-32));
#21335=DIRECTION('',(0.,-1.,-1.E-15));
#21336=DIRECTION('',(1.,0.,0.));
#21337=DIRECTION('center_axis',(0.866025403784448,4.99999999999983E-16,
-0.499999999999983));
#21338=DIRECTION('ref_axis',(-0.499999999999983,8.66025403784449E-16,-0.866025403784448));
#21339=DIRECTION('',(0.499999999999983,-8.96640562630007E-16,0.866025403784448));
#21340=DIRECTION('',(0.,-1.,-1.E-15));
#21341=DIRECTION('',(0.499999999999983,-8.96640562630007E-16,0.866025403784448));
#21342=DIRECTION('',(-0.499999999999983,8.66025403784449E-16,-0.866025403784448));
#21343=DIRECTION('center_axis',(0.866025403784448,-4.99999999999983E-16,
0.499999999999983));
#21344=DIRECTION('ref_axis',(-2.30491487599793E-32,-1.,-1.E-15));
#21345=DIRECTION('',(-0.499999999999983,-8.3541024493889E-16,0.866025403784448));
#21346=DIRECTION('',(-0.499999999999983,-8.3541024493889E-16,0.866025403784448));
#21347=DIRECTION('',(-0.499999999999983,-8.3541024493889E-16,0.866025403784448));
#21348=DIRECTION('',(0.499999999999983,8.66025403784449E-16,-0.866025403784448));
#21349=DIRECTION('center_axis',(0.,1.,1.E-15));
#21350=DIRECTION('ref_axis',(-1.,0.,0.));
#21351=DIRECTION('center_axis',(0.,1.,1.E-15));
#21352=DIRECTION('ref_axis',(-1.,0.,0.));
#21353=DIRECTION('center_axis',(0.,1.,1.E-15));
#21354=DIRECTION('ref_axis',(-1.,0.,0.));
#21355=DIRECTION('center_axis',(0.,1.,1.E-15));
#21356=DIRECTION('ref_axis',(-1.,0.,0.));
#62779=CARTESIAN_POINT('',(0.,0.,0.));
#62780=CARTESIAN_POINT('Origin',(-2.00081E-7,47.4,24.));
#62781=CARTESIAN_POINT('',(-2.00080999566319E-7,48.8433756729741,24.));
#62782=CARTESIAN_POINT('',(-2.00081E-7,47.4,21.5));
#62783=CARTESIAN_POINT('',(-2.00080999693838E-7,47.4,21.5));
#62784=CARTESIAN_POINT('',(2.16506330938012,47.4,22.75));
#62785=CARTESIAN_POINT('Origin',(-2.00081E-7,47.4,24.));
#62786=CARTESIAN_POINT('',(2.16506330938012,47.4,25.25));
#62787=CARTESIAN_POINT('Origin',(-2.00081E-7,47.4,24.));
#62788=CARTESIAN_POINT('',(-2.00081E-7,47.4,26.5));
#62789=CARTESIAN_POINT('Origin',(-2.00081E-7,47.4,24.));
#62790=CARTESIAN_POINT('',(-2.16506370954212,47.4,25.25));
#62791=CARTESIAN_POINT('Origin',(-2.00081E-7,47.4,24.));
#62792=CARTESIAN_POINT('',(-2.16506370954212,47.4,22.75));
#62793=CARTESIAN_POINT('Origin',(-2.00081E-7,47.4,24.));
#62794=CARTESIAN_POINT('Origin',(-2.00081E-7,47.4,24.));
#62795=CARTESIAN_POINT('Origin',(-2.00081E-7,44.4,24.));
#62796=CARTESIAN_POINT('',(1.42982496405621,44.4,26.5));
#62797=CARTESIAN_POINT('',(-1.42982536421821,44.4,26.5));
#62798=CARTESIAN_POINT('Ctrl Pts',(-1.42982536421823,44.4,26.5));
#62799=CARTESIAN_POINT('Ctrl Pts',(-2.00081006429542E-7,44.8098385035873,
26.5));
#62800=CARTESIAN_POINT('Ctrl Pts',(1.42982496405621,44.4,26.5));
#62801=CARTESIAN_POINT('Origin',(-2.00081E-7,44.4,24.));
#62802=CARTESIAN_POINT('Origin',(-2.00081E-7,45.0000000000001,24.));
#62803=CARTESIAN_POINT('',(-2.00080999461155E-7,44.4,19.6));
#62804=CARTESIAN_POINT('Origin',(-2.00081E-7,44.4,24.));
#62805=CARTESIAN_POINT('',(-2.00080999387677E-7,45.,19.));
#62806=CARTESIAN_POINT('Origin',(-2.00080999461155E-7,45.0000000000001,
19.6000000000001));
#62807=CARTESIAN_POINT('',(-2.00080999387677E-7,45.,29.));
#62808=CARTESIAN_POINT('Origin',(-2.00081E-7,45.,24.));
#62809=CARTESIAN_POINT('Origin',(-2.00081E-7,45.,24.));
#62810=CARTESIAN_POINT('Origin',(-2.00081E-7,62.4,24.));
#62811=CARTESIAN_POINT('',(-2.00081000612323E-7,50.4,29.));
#62812=CARTESIAN_POINT('',(-2.00081000612323E-7,62.4,29.));
#62813=CARTESIAN_POINT('Origin',(-2.00081E-7,50.4,24.));
#62814=CARTESIAN_POINT('Origin',(-2.00081E-7,51.0799999999998,24.));
#62815=CARTESIAN_POINT('',(-2.00080999630898E-7,50.9976569609204,20.9860500453614));
#62816=CARTESIAN_POINT('Origin',(-2.00081E-7,50.9976569609204,24.));
#62817=CARTESIAN_POINT('',(-2.00080999632606E-7,51.0799999999998,21.));
#62818=CARTESIAN_POINT('Origin',(-2.0008099960199E-7,51.0799999999998,20.7500000000018));
#62819=CARTESIAN_POINT('',(-2.00080999632606E-7,51.0799999999998,27.));
#62820=CARTESIAN_POINT('Origin',(-2.00081E-7,51.0799999999998,24.));
#62821=CARTESIAN_POINT('Origin',(-2.00081E-7,51.0799999999998,24.));
#62822=CARTESIAN_POINT('Origin',(-2.00081E-7,62.4,24.));
#62823=CARTESIAN_POINT('',(-2.00081000367394E-7,61.7865,27.));
#62824=CARTESIAN_POINT('',(-2.00081000367394E-7,62.4,27.));
#62825=CARTESIAN_POINT('',(-2.00081000367394E-7,61.7865,21.));
#62826=CARTESIAN_POINT('Origin',(-2.00081E-7,61.7865,24.));
#62827=CARTESIAN_POINT('Origin',(-2.00081E-7,61.7865,24.));
#62828=CARTESIAN_POINT('Origin',(-2.00081E-7,50.6499999999998,24.));
#62829=CARTESIAN_POINT('',(-2.0008099958362E-7,50.4,20.6));
#62830=CARTESIAN_POINT('Origin',(-2.00081E-7,50.4,24.));
#62831=CARTESIAN_POINT('',(-2.00080999612528E-7,50.5676569609204,20.8360500453614));
#62832=CARTESIAN_POINT('Origin',(-2.0008099958362E-7,50.6499999999998,20.6000000000001));
#62833=CARTESIAN_POINT('Origin',(-2.00081E-7,50.5676569609204,24.));
#62834=CARTESIAN_POINT('Origin',(-2.00081E-7,61.7865,24.));
#62835=CARTESIAN_POINT('',(-2.00080999707738E-7,62.4,21.6135));
#62836=CARTESIAN_POINT('',(-2.00080999632606E-7,61.7865,21.));
#62837=CARTESIAN_POINT('Origin',(-2.00081E-7,62.4,24.));
#62838=CARTESIAN_POINT('Origin',(-2.00081E-7,50.9976569609204,24.));
#62839=CARTESIAN_POINT('',(-2.00080999630898E-7,50.9976569609204,20.9860500453614));
#62840=CARTESIAN_POINT('Origin',(-2.00081E-7,62.4,21.6135));
#62841=CARTESIAN_POINT('Origin',(-2.00081E-7,44.4,24.));
#62842=CARTESIAN_POINT('',(-1.42982536421821,44.4,21.5));
#62843=CARTESIAN_POINT('',(1.42982496405621,44.4,21.5));
#62844=CARTESIAN_POINT('Ctrl Pts',(-1.42982536421821,44.4,21.5));
#62845=CARTESIAN_POINT('Ctrl Pts',(-2.00081004042563E-7,44.8098385035873,
21.5));
#62846=CARTESIAN_POINT('Ctrl Pts',(1.4298249640562,44.4,21.5));
#62847=CARTESIAN_POINT('Origin',(-2.00081E-7,44.4,24.));
#62848=CARTESIAN_POINT('Origin',(-2.00081E-7,44.4,24.));
#62849=CARTESIAN_POINT('',(-2.8799762916107,44.4,23.9882649151131));
#62850=CARTESIAN_POINT('',(-1.45015112747354,44.4,21.511735084887));
#62851=CARTESIAN_POINT('Ctrl Pts',(-2.87997629161071,44.4,23.9882649151131));
#62852=CARTESIAN_POINT('Ctrl Pts',(-2.16506370954213,44.8098385035873,22.7500000000001));
#62853=CARTESIAN_POINT('Ctrl Pts',(-1.45015112747356,44.4,21.511735084887));
#62854=CARTESIAN_POINT('Origin',(-2.00081E-7,44.4,24.));
#62855=CARTESIAN_POINT('Origin',(-2.00081E-7,44.4,24.));
#62856=CARTESIAN_POINT('',(1.45015072731155,44.4,21.511735084887));
#62857=CARTESIAN_POINT('',(2.8799758914487,44.4,23.9882649151131));
#62858=CARTESIAN_POINT('Ctrl Pts',(1.45015072731154,44.4,21.511735084887));
#62859=CARTESIAN_POINT('Ctrl Pts',(2.16506330938013,44.8098385035873,22.75));
#62860=CARTESIAN_POINT('Ctrl Pts',(2.8799758914487,44.4,23.9882649151131));
#62861=CARTESIAN_POINT('Origin',(-2.00081E-7,44.4,24.));
#62862=CARTESIAN_POINT('Origin',(-2.500000200081,47.4,24.));
#62863=CARTESIAN_POINT('',(-1.4433758730551,47.4,26.5));
#62864=CARTESIAN_POINT('',(-2.8867515460291,47.4,24.));
#62865=CARTESIAN_POINT('',(-1.4433758730551,47.4,26.5));
#62866=CARTESIAN_POINT('Origin',(-2.00081E-7,44.4,24.));
#62867=CARTESIAN_POINT('',(-1.45015112747355,44.4,26.488264915113));
#62868=CARTESIAN_POINT('',(-2.8799762916107,44.4,24.0117350848869));
#62869=CARTESIAN_POINT('Ctrl Pts',(-1.45015112747355,44.4,26.488264915113));
#62870=CARTESIAN_POINT('Ctrl Pts',(-2.16506370954212,44.8098385035873,25.25));
#62871=CARTESIAN_POINT('Ctrl Pts',(-2.8799762916107,44.4,24.0117350848869));
#62872=CARTESIAN_POINT('Origin',(-2.00081E-7,44.4,24.));
#62873=CARTESIAN_POINT('Origin',(-2.00081E-7,44.4,24.));
#62874=CARTESIAN_POINT('',(2.8799758914487,44.4,24.0117350848869));
#62875=CARTESIAN_POINT('',(1.45015072731154,44.4,26.488264915113));
#62876=CARTESIAN_POINT('Ctrl Pts',(2.8799758914487,44.4,24.0117350848869));
#62877=CARTESIAN_POINT('Ctrl Pts',(2.16506330938012,44.8098385035873,25.25));
#62878=CARTESIAN_POINT('Ctrl Pts',(1.45015072731155,44.4,26.488264915113));
#62879=CARTESIAN_POINT('Origin',(-2.00081E-7,44.4,24.));
#62880=CARTESIAN_POINT('Origin',(-2.500000200081,47.4,24.));
#62881=CARTESIAN_POINT('',(1.4433754728931,47.4,26.5));
#62882=CARTESIAN_POINT('',(-1.4433758730551,47.4,26.5));
#62883=CARTESIAN_POINT('',(1.4433754728931,47.4,26.5));
#62884=CARTESIAN_POINT('Origin',(-2.500000200081,47.4,24.));
#62885=CARTESIAN_POINT('',(2.8867511458671,47.4,24.));
#62886=CARTESIAN_POINT('',(1.4433754728931,47.4,26.5));
#62887=CARTESIAN_POINT('',(2.8867511458671,47.4,24.));
#62888=CARTESIAN_POINT('Origin',(-2.00081E-7,50.4,19.));
#62889=CARTESIAN_POINT('Origin',(-1.4433758730551,47.4,26.5));
#62890=CARTESIAN_POINT('',(-1.4433758730551,44.4,26.5));
#62891=CARTESIAN_POINT('',(-1.4433758730551,44.4,26.5));
#62892=CARTESIAN_POINT('',(-1.4433758730551,47.4,26.5));
#62893=CARTESIAN_POINT('',(1.4433754728931,44.4,26.5));
#62894=CARTESIAN_POINT('',(1.4433754728931,47.4,26.5));
#62895=CARTESIAN_POINT('',(-2.00081E-7,44.4,26.5));
#62896=CARTESIAN_POINT('Origin',(1.4433754728931,47.4,26.5));
#62897=CARTESIAN_POINT('',(1.4433754728931,44.4,26.5));
#62898=CARTESIAN_POINT('',(2.8867511458671,44.4,24.));
#62899=CARTESIAN_POINT('',(2.8867511458671,47.4,24.));
#62900=CARTESIAN_POINT('',(2.16506330938012,44.4,25.25));
#62901=CARTESIAN_POINT('Origin',(2.8867511458671,47.4,24.));
#62902=CARTESIAN_POINT('',(2.8867511458671,44.4,24.));
#62903=CARTESIAN_POINT('',(1.4433754728931,47.4,21.5));
#62904=CARTESIAN_POINT('',(2.8867511458671,47.4,24.));
#62905=CARTESIAN_POINT('',(1.4433754728931,44.4,21.5));
#62906=CARTESIAN_POINT('',(1.4433754728931,47.4,21.5));
#62907=CARTESIAN_POINT('',(2.16506330938012,44.4,22.75));
#62908=CARTESIAN_POINT('Origin',(1.4433754728931,47.4,21.5));
#62909=CARTESIAN_POINT('',(1.4433754728931,44.4,21.5));
#62910=CARTESIAN_POINT('',(1.4433754728931,47.4,21.5));
#62911=CARTESIAN_POINT('',(-1.4433758730551,47.4,21.5));
#62912=CARTESIAN_POINT('',(1.4433754728931,47.4,21.5));
#62913=CARTESIAN_POINT('',(-1.4433758730551,44.4,21.5));
#62914=CARTESIAN_POINT('',(-1.4433758730551,47.4,21.5));
#62915=CARTESIAN_POINT('',(-2.00081E-7,44.4,21.5));
#62916=CARTESIAN_POINT('Origin',(-2.8867515460291,47.4,24.));
#62917=CARTESIAN_POINT('',(-2.8867515460291,44.4,24.));
#62918=CARTESIAN_POINT('',(-2.8867515460291,44.4,24.));
#62919=CARTESIAN_POINT('',(-2.8867515460291,47.4,24.));
#62920=CARTESIAN_POINT('',(-2.8867515460291,47.4,24.));
#62921=CARTESIAN_POINT('',(-2.8867515460291,47.4,24.));
#62922=CARTESIAN_POINT('',(-2.16506370954212,44.4,25.25));
#62923=CARTESIAN_POINT('Origin',(-1.4433758730551,47.4,21.5));
#62924=CARTESIAN_POINT('',(-1.4433758730551,44.4,21.5));
#62925=CARTESIAN_POINT('',(-1.4433758730551,47.4,21.5));
#62926=CARTESIAN_POINT('',(-1.4433758730551,47.4,21.5));
#62927=CARTESIAN_POINT('',(-2.16506370954212,44.4,22.75));
#62928=CARTESIAN_POINT('Origin',(-2.500000200081,47.4,24.));
#62929=CARTESIAN_POINT('Origin',(-2.500000200081,47.4,24.));
#62930=CARTESIAN_POINT('Origin',(-2.00081E-7,44.4,24.));
#62931=CARTESIAN_POINT('Origin',(-2.500000200081,47.4,24.));
#62959=UNCERTAINTY_MEASURE_WITH_UNIT(LENGTH_MEASURE(0.01),#62975,
'DISTANCE_ACCURACY_VALUE',
'Maximum model space distance between geometric entities at asserted c
onnectivities');
#62960=UNCERTAINTY_MEASURE_WITH_UNIT(LENGTH_MEASURE(0.01),#62975,
'DISTANCE_ACCURACY_VALUE',
'Maximum model space distance between geometric entities at asserted c
onnectivities');
#62973=(
GEOMETRIC_REPRESENTATION_CONTEXT(3)
GLOBAL_UNCERTAINTY_ASSIGNED_CONTEXT((#62959))
GLOBAL_UNIT_ASSIGNED_CONTEXT((#62975,#62977,#62978))
REPRESENTATION_CONTEXT('','3D')
);
#62974=(
GEOMETRIC_REPRESENTATION_CONTEXT(3)
GLOBAL_UNCERTAINTY_ASSIGNED_CONTEXT((#62960))
GLOBAL_UNIT_ASSIGNED_CONTEXT((#62975,#62977,#62978))
REPRESENTATION_CONTEXT('','3D')
);
#62975=(
LENGTH_UNIT()
NAMED_UNIT(*)
SI_UNIT(.MILLI.,.METRE.)
);
#62977=(
NAMED_UNIT(*)
PLANE_ANGLE_UNIT()
SI_UNIT($,.RADIAN.)
);
#62978=(
NAMED_UNIT(*)
SI_UNIT($,.STERADIAN.)
SOLID_ANGLE_UNIT()
);
#62991=SHAPE_DEFINITION_REPRESENTATION(#63004,#63032);
#63004=PRODUCT_DEFINITION_SHAPE('',$,#63046);
#63032=SHAPE_REPRESENTATION('',(#16884),#62973);
#63033=PRODUCT_DEFINITION_CONTEXT('part definition',#63074,'design');
#63046=PRODUCT_DEFINITION('DIN 912 M6x12','DIN 912 M6x12',#63059,#63033);
#63059=PRODUCT_DEFINITION_FORMATION('',$,#63088);
#63074=APPLICATION_CONTEXT(
'Core Data for Automotive Mechanical Design Process');
#63075=PRODUCT_CONTEXT('part definition',#63074,'mechanical');
#63088=PRODUCT('DIN 912 M6x12','DIN 912 M6x12',$,(#63075));
#63090=PRESENTATION_STYLE_ASSIGNMENT((#63092));
#63092=SURFACE_STYLE_USAGE(.BOTH.,#63094);
#63094=SURFACE_SIDE_STYLE('',(#63096));
#63096=SURFACE_STYLE_FILL_AREA(#63098);
#63098=FILL_AREA_STYLE('Opaque(202,209,238)',(#63100));
#63100=FILL_AREA_STYLE_COLOUR('Opaque(202,209,238)',#63102);
#63102=COLOUR_RGB('Opaque(202,209,238)', 0.66274510, 0.83137255, 0.94901961);
ENDSEC;
END-ISO-10303-21;
